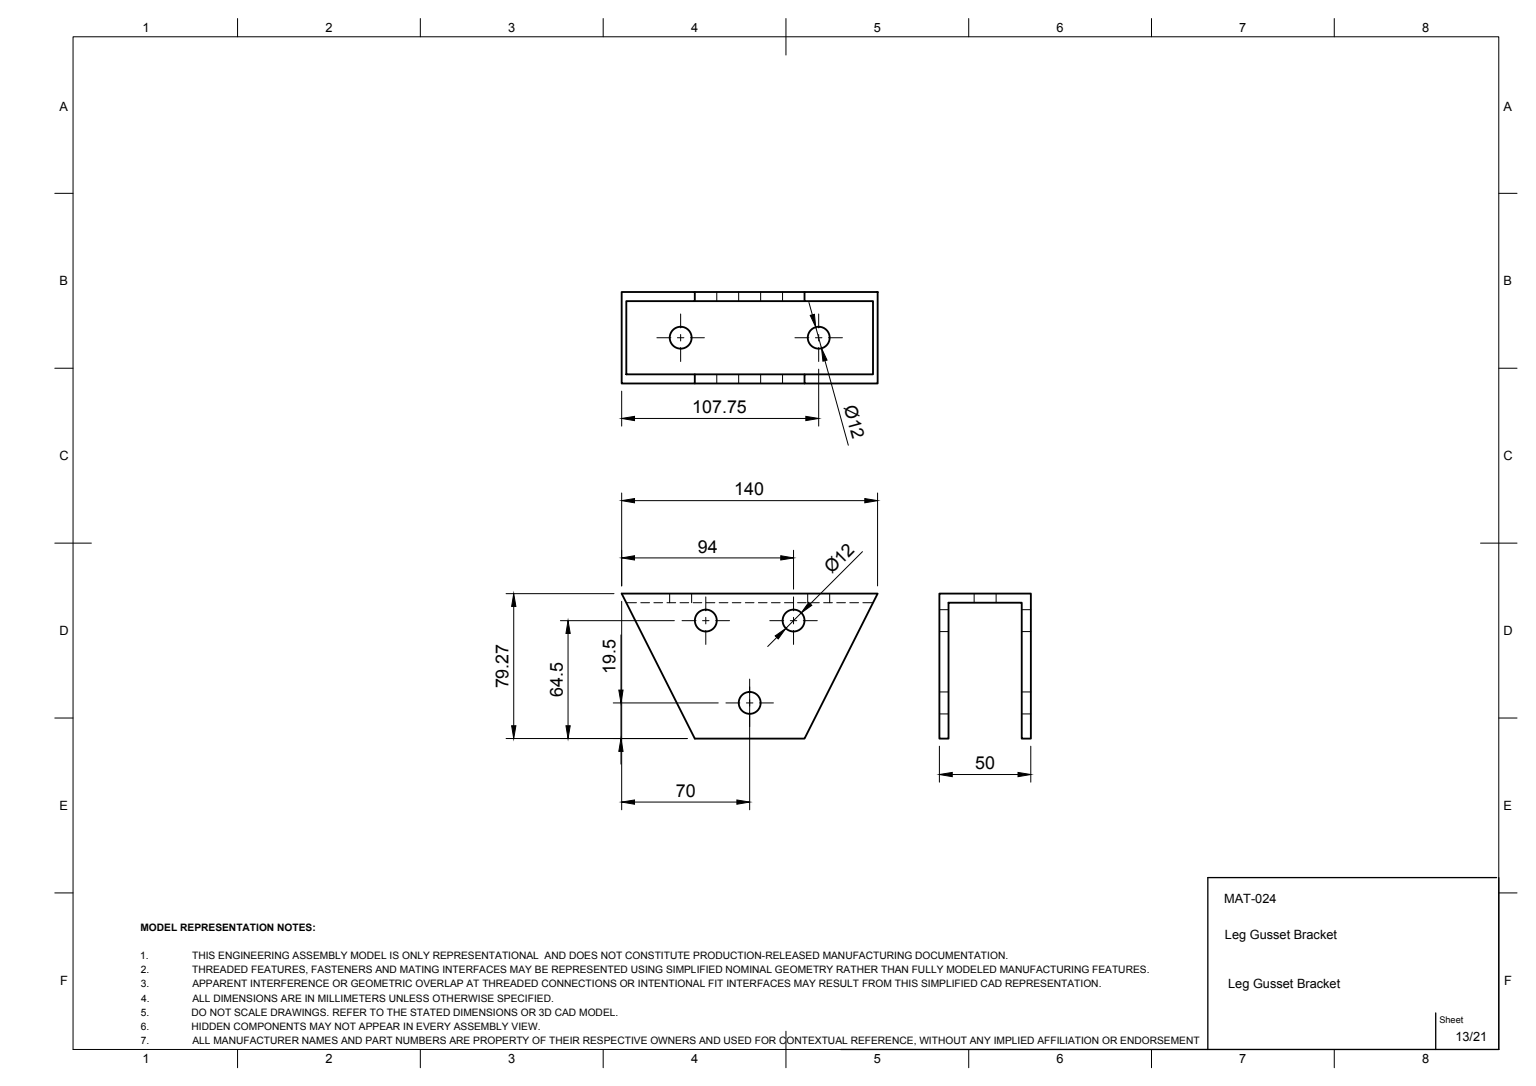
ISO-10303-21;
HEADER;
/* Generated by software containing ST-Developer
 * from STEP Tools, Inc. (www.steptools.com) 
 */

FILE_DESCRIPTION(
/* description */ ('STEP AP214'),
/* implementation_level */ '2;1');

FILE_NAME(
/* name */ 'Leg Gusset Bracket.step',
/* time_stamp */ '2026-11-14T06:34:07-08:00',
/* author */ (''),
/* organization */ (''),
/* preprocessor_version */ 'ST-DEVELOPER v20.2',
/* originating_system */ 'Autodesk Translation Framework v15.17.0.0',
/* authorisation */ '');

FILE_SCHEMA (('AUTOMOTIVE_DESIGN { 1 0 10303 214 3 1 1 }'));
ENDSEC;

DATA;
#10=MECHANICAL_DESIGN_GEOMETRIC_PRESENTATION_REPRESENTATION('',(#7320),#310623);
#7235=SHAPE_REPRESENTATION_RELATIONSHIP('SRR','None',#310909,#7252);
#7252=ADVANCED_BREP_SHAPE_REPRESENTATION('',(#7387),#310618);
#7320=STYLED_ITEM('',(#311004),#7387);
#7387=MANIFOLD_SOLID_BREP('Body1',#93771);
#7676=FACE_BOUND('',#20280,.T.);
#7677=FACE_BOUND('',#20281,.T.);
#7678=FACE_BOUND('',#20283,.T.);
#7679=FACE_BOUND('',#20284,.T.);
#7680=FACE_BOUND('',#20285,.T.);
#7681=FACE_BOUND('',#20287,.T.);
#7682=FACE_BOUND('',#20288,.T.);
#7683=FACE_BOUND('',#20289,.T.);
#7684=FACE_BOUND('',#20291,.T.);
#7685=FACE_BOUND('',#20292,.T.);
#7686=FACE_BOUND('',#20293,.T.);
#7687=FACE_BOUND('',#20295,.T.);
#7688=FACE_BOUND('',#20296,.T.);
#7689=FACE_BOUND('',#20298,.T.);
#7690=FACE_BOUND('',#20299,.T.);
#7691=FACE_BOUND('',#20300,.T.);
#8632=PLANE('',#104587);
#8633=PLANE('',#104588);
#8634=PLANE('',#104589);
#8635=PLANE('',#104590);
#8636=PLANE('',#104591);
#8637=PLANE('',#104592);
#8638=PLANE('',#104593);
#8639=PLANE('',#104594);
#8640=PLANE('',#104595);
#8641=PLANE('',#104596);
#14243=FACE_OUTER_BOUND('',#20267,.T.);
#14244=FACE_OUTER_BOUND('',#20268,.T.);
#14245=FACE_OUTER_BOUND('',#20269,.T.);
#14246=FACE_OUTER_BOUND('',#20270,.T.);
#14247=FACE_OUTER_BOUND('',#20271,.T.);
#14248=FACE_OUTER_BOUND('',#20272,.T.);
#14249=FACE_OUTER_BOUND('',#20273,.T.);
#14250=FACE_OUTER_BOUND('',#20274,.T.);
#14251=FACE_OUTER_BOUND('',#20275,.T.);
#14252=FACE_OUTER_BOUND('',#20276,.T.);
#14253=FACE_OUTER_BOUND('',#20277,.T.);
#14254=FACE_OUTER_BOUND('',#20278,.T.);
#14255=FACE_OUTER_BOUND('',#20279,.T.);
#14256=FACE_OUTER_BOUND('',#20282,.T.);
#14257=FACE_OUTER_BOUND('',#20286,.T.);
#14258=FACE_OUTER_BOUND('',#20290,.T.);
#14259=FACE_OUTER_BOUND('',#20294,.T.);
#14260=FACE_OUTER_BOUND('',#20297,.T.);
#20267=EDGE_LOOP('',(#84815,#84816,#84817,#84818));
#20268=EDGE_LOOP('',(#84819,#84820,#84821,#84822));
#20269=EDGE_LOOP('',(#84823,#84824,#84825,#84826));
#20270=EDGE_LOOP('',(#84827,#84828,#84829,#84830));
#20271=EDGE_LOOP('',(#84831,#84832,#84833,#84834));
#20272=EDGE_LOOP('',(#84835,#84836,#84837,#84838));
#20273=EDGE_LOOP('',(#84839,#84840,#84841,#84842));
#20274=EDGE_LOOP('',(#84843,#84844,#84845,#84846));
#20275=EDGE_LOOP('',(#84847,#84848,#84849,#84850,#84851,#84852,#84853,#84854));
#20276=EDGE_LOOP('',(#84855,#84856,#84857,#84858,#84859,#84860,#84861,#84862));
#20277=EDGE_LOOP('',(#84863,#84864,#84865,#84866));
#20278=EDGE_LOOP('',(#84867,#84868,#84869,#84870));
#20279=EDGE_LOOP('',(#84871,#84872,#84873,#84874));
#20280=EDGE_LOOP('',(#84875));
#20281=EDGE_LOOP('',(#84876));
#20282=EDGE_LOOP('',(#84877,#84878,#84879,#84880));
#20283=EDGE_LOOP('',(#84881));
#20284=EDGE_LOOP('',(#84882));
#20285=EDGE_LOOP('',(#84883));
#20286=EDGE_LOOP('',(#84884,#84885,#84886,#84887));
#20287=EDGE_LOOP('',(#84888));
#20288=EDGE_LOOP('',(#84889));
#20289=EDGE_LOOP('',(#84890));
#20290=EDGE_LOOP('',(#84891,#84892,#84893,#84894));
#20291=EDGE_LOOP('',(#84895));
#20292=EDGE_LOOP('',(#84896));
#20293=EDGE_LOOP('',(#84897));
#20294=EDGE_LOOP('',(#84898,#84899,#84900,#84901));
#20295=EDGE_LOOP('',(#84902));
#20296=EDGE_LOOP('',(#84903));
#20297=EDGE_LOOP('',(#84904,#84905,#84906,#84907));
#20298=EDGE_LOOP('',(#84908));
#20299=EDGE_LOOP('',(#84909));
#20300=EDGE_LOOP('',(#84910));
#24640=LINE('',#302816,#28987);
#24641=LINE('',#302822,#28988);
#24642=LINE('',#302828,#28989);
#24643=LINE('',#302834,#28990);
#24644=LINE('',#302840,#28991);
#24645=LINE('',#302846,#28992);
#24646=LINE('',#302852,#28993);
#24647=LINE('',#302858,#28994);
#24648=LINE('',#302863,#28995);
#24649=LINE('',#302865,#28996);
#24650=LINE('',#302867,#28997);
#24651=LINE('',#302869,#28998);
#24652=LINE('',#302871,#28999);
#24653=LINE('',#302873,#29000);
#24654=LINE('',#302875,#29001);
#24655=LINE('',#302876,#29002);
#24656=LINE('',#302880,#29003);
#24657=LINE('',#302882,#29004);
#24658=LINE('',#302884,#29005);
#24659=LINE('',#302886,#29006);
#24660=LINE('',#302888,#29007);
#24661=LINE('',#302890,#29008);
#24662=LINE('',#302892,#29009);
#24663=LINE('',#302893,#29010);
#24664=LINE('',#302895,#29011);
#24665=LINE('',#302896,#29012);
#24666=LINE('',#302898,#29013);
#24667=LINE('',#302899,#29014);
#24668=LINE('',#302901,#29015);
#24669=LINE('',#302902,#29016);
#24670=LINE('',#302906,#29017);
#24671=LINE('',#302908,#29018);
#28987=VECTOR('',#130227,6.00000000000001);
#28988=VECTOR('',#130234,6.00000000000001);
#28989=VECTOR('',#130241,6.00000000000001);
#28990=VECTOR('',#130248,6.00000000000001);
#28991=VECTOR('',#130255,6.00000000000001);
#28992=VECTOR('',#130262,6.00000000000001);
#28993=VECTOR('',#130269,6.00000000000001);
#28994=VECTOR('',#130276,6.00000000000001);
#28995=VECTOR('',#130281,1000.);
#28996=VECTOR('',#130282,1000.);
#28997=VECTOR('',#130283,1000.);
#28998=VECTOR('',#130284,1000.);
#28999=VECTOR('',#130285,1000.);
#29000=VECTOR('',#130286,1000.);
#29001=VECTOR('',#130287,1000.);
#29002=VECTOR('',#130288,1000.);
#29003=VECTOR('',#130291,1000.);
#29004=VECTOR('',#130292,1000.);
#29005=VECTOR('',#130293,1000.);
#29006=VECTOR('',#130294,1000.);
#29007=VECTOR('',#130295,1000.);
#29008=VECTOR('',#130296,1000.);
#29009=VECTOR('',#130297,1000.);
#29010=VECTOR('',#130298,1000.);
#29011=VECTOR('',#130301,1000.);
#29012=VECTOR('',#130302,1000.);
#29013=VECTOR('',#130305,1000.);
#29014=VECTOR('',#130306,1000.);
#29015=VECTOR('',#130309,1000.);
#29016=VECTOR('',#130310,1000.);
#29017=VECTOR('',#130317,1000.);
#29018=VECTOR('',#130320,1000.);
#35041=CIRCLE('',#104564,6.00000000000001);
#35042=CIRCLE('',#104565,6.00000000000001);
#35043=CIRCLE('',#104567,6.00000000000001);
#35044=CIRCLE('',#104568,6.00000000000001);
#35045=CIRCLE('',#104570,5.99999999999999);
#35046=CIRCLE('',#104571,6.00000000000001);
#35047=CIRCLE('',#104573,5.99999999999999);
#35048=CIRCLE('',#104574,6.00000000000001);
#35049=CIRCLE('',#104576,5.99999999999999);
#35050=CIRCLE('',#104577,6.00000000000001);
#35051=CIRCLE('',#104579,6.00000000000001);
#35052=CIRCLE('',#104580,6.00000000000001);
#35053=CIRCLE('',#104582,6.00000000000001);
#35054=CIRCLE('',#104583,6.00000000000001);
#35055=CIRCLE('',#104585,6.00000000000001);
#35056=CIRCLE('',#104586,6.00000000000001);
#43306=VERTEX_POINT('',#302813);
#43307=VERTEX_POINT('',#302815);
#43308=VERTEX_POINT('',#302819);
#43309=VERTEX_POINT('',#302821);
#43310=VERTEX_POINT('',#302825);
#43311=VERTEX_POINT('',#302827);
#43312=VERTEX_POINT('',#302831);
#43313=VERTEX_POINT('',#302833);
#43314=VERTEX_POINT('',#302837);
#43315=VERTEX_POINT('',#302839);
#43316=VERTEX_POINT('',#302843);
#43317=VERTEX_POINT('',#302845);
#43318=VERTEX_POINT('',#302849);
#43319=VERTEX_POINT('',#302851);
#43320=VERTEX_POINT('',#302855);
#43321=VERTEX_POINT('',#302857);
#43322=VERTEX_POINT('',#302861);
#43323=VERTEX_POINT('',#302862);
#43324=VERTEX_POINT('',#302864);
#43325=VERTEX_POINT('',#302866);
#43326=VERTEX_POINT('',#302868);
#43327=VERTEX_POINT('',#302870);
#43328=VERTEX_POINT('',#302872);
#43329=VERTEX_POINT('',#302874);
#43330=VERTEX_POINT('',#302878);
#43331=VERTEX_POINT('',#302879);
#43332=VERTEX_POINT('',#302881);
#43333=VERTEX_POINT('',#302883);
#43334=VERTEX_POINT('',#302885);
#43335=VERTEX_POINT('',#302887);
#43336=VERTEX_POINT('',#302889);
#43337=VERTEX_POINT('',#302891);
#57187=EDGE_CURVE('',#43306,#43306,#35041,.T.);
#57188=EDGE_CURVE('',#43306,#43307,#24640,.T.);
#57189=EDGE_CURVE('',#43307,#43307,#35042,.T.);
#57190=EDGE_CURVE('',#43308,#43308,#35043,.T.);
#57191=EDGE_CURVE('',#43308,#43309,#24641,.T.);
#57192=EDGE_CURVE('',#43309,#43309,#35044,.T.);
#57193=EDGE_CURVE('',#43310,#43310,#35045,.T.);
#57194=EDGE_CURVE('',#43310,#43311,#24642,.T.);
#57195=EDGE_CURVE('',#43311,#43311,#35046,.T.);
#57196=EDGE_CURVE('',#43312,#43312,#35047,.T.);
#57197=EDGE_CURVE('',#43312,#43313,#24643,.T.);
#57198=EDGE_CURVE('',#43313,#43313,#35048,.T.);
#57199=EDGE_CURVE('',#43314,#43314,#35049,.T.);
#57200=EDGE_CURVE('',#43314,#43315,#24644,.T.);
#57201=EDGE_CURVE('',#43315,#43315,#35050,.T.);
#57202=EDGE_CURVE('',#43316,#43316,#35051,.T.);
#57203=EDGE_CURVE('',#43316,#43317,#24645,.T.);
#57204=EDGE_CURVE('',#43317,#43317,#35052,.T.);
#57205=EDGE_CURVE('',#43318,#43318,#35053,.T.);
#57206=EDGE_CURVE('',#43318,#43319,#24646,.T.);
#57207=EDGE_CURVE('',#43319,#43319,#35054,.T.);
#57208=EDGE_CURVE('',#43320,#43320,#35055,.T.);
#57209=EDGE_CURVE('',#43320,#43321,#24647,.T.);
#57210=EDGE_CURVE('',#43321,#43321,#35056,.T.);
#57211=EDGE_CURVE('',#43322,#43323,#24648,.T.);
#57212=EDGE_CURVE('',#43323,#43324,#24649,.T.);
#57213=EDGE_CURVE('',#43324,#43325,#24650,.T.);
#57214=EDGE_CURVE('',#43326,#43325,#24651,.T.);
#57215=EDGE_CURVE('',#43327,#43326,#24652,.T.);
#57216=EDGE_CURVE('',#43327,#43328,#24653,.T.);
#57217=EDGE_CURVE('',#43328,#43329,#24654,.T.);
#57218=EDGE_CURVE('',#43329,#43322,#24655,.T.);
#57219=EDGE_CURVE('',#43330,#43331,#24656,.T.);
#57220=EDGE_CURVE('',#43330,#43332,#24657,.T.);
#57221=EDGE_CURVE('',#43332,#43333,#24658,.T.);
#57222=EDGE_CURVE('',#43333,#43334,#24659,.T.);
#57223=EDGE_CURVE('',#43335,#43334,#24660,.T.);
#57224=EDGE_CURVE('',#43335,#43336,#24661,.T.);
#57225=EDGE_CURVE('',#43336,#43337,#24662,.T.);
#57226=EDGE_CURVE('',#43331,#43337,#24663,.T.);
#57227=EDGE_CURVE('',#43324,#43330,#24664,.T.);
#57228=EDGE_CURVE('',#43325,#43331,#24665,.T.);
#57229=EDGE_CURVE('',#43334,#43329,#24666,.T.);
#57230=EDGE_CURVE('',#43328,#43335,#24667,.T.);
#57231=EDGE_CURVE('',#43337,#43326,#24668,.T.);
#57232=EDGE_CURVE('',#43336,#43327,#24669,.T.);
#57233=EDGE_CURVE('',#43323,#43332,#24670,.T.);
#57234=EDGE_CURVE('',#43322,#43333,#24671,.T.);
#84815=ORIENTED_EDGE('',*,*,#57187,.F.);
#84816=ORIENTED_EDGE('',*,*,#57188,.T.);
#84817=ORIENTED_EDGE('',*,*,#57189,.T.);
#84818=ORIENTED_EDGE('',*,*,#57188,.F.);
#84819=ORIENTED_EDGE('',*,*,#57190,.F.);
#84820=ORIENTED_EDGE('',*,*,#57191,.T.);
#84821=ORIENTED_EDGE('',*,*,#57192,.T.);
#84822=ORIENTED_EDGE('',*,*,#57191,.F.);
#84823=ORIENTED_EDGE('',*,*,#57193,.T.);
#84824=ORIENTED_EDGE('',*,*,#57194,.T.);
#84825=ORIENTED_EDGE('',*,*,#57195,.T.);
#84826=ORIENTED_EDGE('',*,*,#57194,.F.);
#84827=ORIENTED_EDGE('',*,*,#57196,.T.);
#84828=ORIENTED_EDGE('',*,*,#57197,.T.);
#84829=ORIENTED_EDGE('',*,*,#57198,.T.);
#84830=ORIENTED_EDGE('',*,*,#57197,.F.);
#84831=ORIENTED_EDGE('',*,*,#57199,.T.);
#84832=ORIENTED_EDGE('',*,*,#57200,.T.);
#84833=ORIENTED_EDGE('',*,*,#57201,.T.);
#84834=ORIENTED_EDGE('',*,*,#57200,.F.);
#84835=ORIENTED_EDGE('',*,*,#57202,.F.);
#84836=ORIENTED_EDGE('',*,*,#57203,.T.);
#84837=ORIENTED_EDGE('',*,*,#57204,.T.);
#84838=ORIENTED_EDGE('',*,*,#57203,.F.);
#84839=ORIENTED_EDGE('',*,*,#57205,.F.);
#84840=ORIENTED_EDGE('',*,*,#57206,.T.);
#84841=ORIENTED_EDGE('',*,*,#57207,.T.);
#84842=ORIENTED_EDGE('',*,*,#57206,.F.);
#84843=ORIENTED_EDGE('',*,*,#57208,.F.);
#84844=ORIENTED_EDGE('',*,*,#57209,.T.);
#84845=ORIENTED_EDGE('',*,*,#57210,.T.);
#84846=ORIENTED_EDGE('',*,*,#57209,.F.);
#84847=ORIENTED_EDGE('',*,*,#57211,.T.);
#84848=ORIENTED_EDGE('',*,*,#57212,.T.);
#84849=ORIENTED_EDGE('',*,*,#57213,.T.);
#84850=ORIENTED_EDGE('',*,*,#57214,.F.);
#84851=ORIENTED_EDGE('',*,*,#57215,.F.);
#84852=ORIENTED_EDGE('',*,*,#57216,.T.);
#84853=ORIENTED_EDGE('',*,*,#57217,.T.);
#84854=ORIENTED_EDGE('',*,*,#57218,.T.);
#84855=ORIENTED_EDGE('',*,*,#57219,.F.);
#84856=ORIENTED_EDGE('',*,*,#57220,.T.);
#84857=ORIENTED_EDGE('',*,*,#57221,.T.);
#84858=ORIENTED_EDGE('',*,*,#57222,.T.);
#84859=ORIENTED_EDGE('',*,*,#57223,.F.);
#84860=ORIENTED_EDGE('',*,*,#57224,.T.);
#84861=ORIENTED_EDGE('',*,*,#57225,.T.);
#84862=ORIENTED_EDGE('',*,*,#57226,.F.);
#84863=ORIENTED_EDGE('',*,*,#57213,.F.);
#84864=ORIENTED_EDGE('',*,*,#57227,.T.);
#84865=ORIENTED_EDGE('',*,*,#57219,.T.);
#84866=ORIENTED_EDGE('',*,*,#57228,.F.);
#84867=ORIENTED_EDGE('',*,*,#57223,.T.);
#84868=ORIENTED_EDGE('',*,*,#57229,.T.);
#84869=ORIENTED_EDGE('',*,*,#57217,.F.);
#84870=ORIENTED_EDGE('',*,*,#57230,.T.);
#84871=ORIENTED_EDGE('',*,*,#57231,.F.);
#84872=ORIENTED_EDGE('',*,*,#57225,.F.);
#84873=ORIENTED_EDGE('',*,*,#57232,.T.);
#84874=ORIENTED_EDGE('',*,*,#57215,.T.);
#84875=ORIENTED_EDGE('',*,*,#57187,.T.);
#84876=ORIENTED_EDGE('',*,*,#57190,.T.);
#84877=ORIENTED_EDGE('',*,*,#57216,.F.);
#84878=ORIENTED_EDGE('',*,*,#57232,.F.);
#84879=ORIENTED_EDGE('',*,*,#57224,.F.);
#84880=ORIENTED_EDGE('',*,*,#57230,.F.);
#84881=ORIENTED_EDGE('',*,*,#57202,.T.);
#84882=ORIENTED_EDGE('',*,*,#57205,.T.);
#84883=ORIENTED_EDGE('',*,*,#57208,.T.);
#84884=ORIENTED_EDGE('',*,*,#57214,.T.);
#84885=ORIENTED_EDGE('',*,*,#57228,.T.);
#84886=ORIENTED_EDGE('',*,*,#57226,.T.);
#84887=ORIENTED_EDGE('',*,*,#57231,.T.);
#84888=ORIENTED_EDGE('',*,*,#57195,.F.);
#84889=ORIENTED_EDGE('',*,*,#57198,.F.);
#84890=ORIENTED_EDGE('',*,*,#57201,.F.);
#84891=ORIENTED_EDGE('',*,*,#57233,.T.);
#84892=ORIENTED_EDGE('',*,*,#57220,.F.);
#84893=ORIENTED_EDGE('',*,*,#57227,.F.);
#84894=ORIENTED_EDGE('',*,*,#57212,.F.);
#84895=ORIENTED_EDGE('',*,*,#57193,.F.);
#84896=ORIENTED_EDGE('',*,*,#57196,.F.);
#84897=ORIENTED_EDGE('',*,*,#57199,.F.);
#84898=ORIENTED_EDGE('',*,*,#57234,.T.);
#84899=ORIENTED_EDGE('',*,*,#57221,.F.);
#84900=ORIENTED_EDGE('',*,*,#57233,.F.);
#84901=ORIENTED_EDGE('',*,*,#57211,.F.);
#84902=ORIENTED_EDGE('',*,*,#57189,.F.);
#84903=ORIENTED_EDGE('',*,*,#57192,.F.);
#84904=ORIENTED_EDGE('',*,*,#57229,.F.);
#84905=ORIENTED_EDGE('',*,*,#57222,.F.);
#84906=ORIENTED_EDGE('',*,*,#57234,.F.);
#84907=ORIENTED_EDGE('',*,*,#57218,.F.);
#84908=ORIENTED_EDGE('',*,*,#57204,.F.);
#84909=ORIENTED_EDGE('',*,*,#57207,.F.);
#84910=ORIENTED_EDGE('',*,*,#57210,.F.);
#87900=CYLINDRICAL_SURFACE('',#104563,6.00000000000001);
#87901=CYLINDRICAL_SURFACE('',#104566,6.00000000000001);
#87902=CYLINDRICAL_SURFACE('',#104569,6.00000000000001);
#87903=CYLINDRICAL_SURFACE('',#104572,6.00000000000001);
#87904=CYLINDRICAL_SURFACE('',#104575,6.00000000000001);
#87905=CYLINDRICAL_SURFACE('',#104578,6.00000000000001);
#87906=CYLINDRICAL_SURFACE('',#104581,6.00000000000001);
#87907=CYLINDRICAL_SURFACE('',#104584,6.00000000000001);
#93522=ADVANCED_FACE('',(#14243),#87900,.F.);
#93523=ADVANCED_FACE('',(#14244),#87901,.F.);
#93524=ADVANCED_FACE('',(#14245),#87902,.F.);
#93525=ADVANCED_FACE('',(#14246),#87903,.F.);
#93526=ADVANCED_FACE('',(#14247),#87904,.F.);
#93527=ADVANCED_FACE('',(#14248),#87905,.F.);
#93528=ADVANCED_FACE('',(#14249),#87906,.F.);
#93529=ADVANCED_FACE('',(#14250),#87907,.F.);
#93530=ADVANCED_FACE('',(#14251),#8632,.T.);
#93531=ADVANCED_FACE('',(#14252),#8633,.T.);
#93532=ADVANCED_FACE('',(#14253),#8634,.T.);
#93533=ADVANCED_FACE('',(#14254),#8635,.T.);
#93534=ADVANCED_FACE('',(#14255,#7676,#7677),#8636,.T.);
#93535=ADVANCED_FACE('',(#14256,#7678,#7679,#7680),#8637,.T.);
#93536=ADVANCED_FACE('',(#14257,#7681,#7682,#7683),#8638,.F.);
#93537=ADVANCED_FACE('',(#14258,#7684,#7685,#7686),#8639,.T.);
#93538=ADVANCED_FACE('',(#14259,#7687,#7688),#8640,.T.);
#93539=ADVANCED_FACE('',(#14260,#7689,#7690,#7691),#8641,.T.);
#93771=CLOSED_SHELL('',(#93522,#93523,#93524,#93525,#93526,#93527,#93528,
#93529,#93530,#93531,#93532,#93533,#93534,#93535,#93536,#93537,#93538,#93539));
#104562=AXIS2_PLACEMENT_3D('',#302811,#130221,#130222);
#104563=AXIS2_PLACEMENT_3D('',#302812,#130223,#130224);
#104564=AXIS2_PLACEMENT_3D('',#302814,#130225,#130226);
#104565=AXIS2_PLACEMENT_3D('',#302817,#130228,#130229);
#104566=AXIS2_PLACEMENT_3D('',#302818,#130230,#130231);
#104567=AXIS2_PLACEMENT_3D('',#302820,#130232,#130233);
#104568=AXIS2_PLACEMENT_3D('',#302823,#130235,#130236);
#104569=AXIS2_PLACEMENT_3D('',#302824,#130237,#130238);
#104570=AXIS2_PLACEMENT_3D('',#302826,#130239,#130240);
#104571=AXIS2_PLACEMENT_3D('',#302829,#130242,#130243);
#104572=AXIS2_PLACEMENT_3D('',#302830,#130244,#130245);
#104573=AXIS2_PLACEMENT_3D('',#302832,#130246,#130247);
#104574=AXIS2_PLACEMENT_3D('',#302835,#130249,#130250);
#104575=AXIS2_PLACEMENT_3D('',#302836,#130251,#130252);
#104576=AXIS2_PLACEMENT_3D('',#302838,#130253,#130254);
#104577=AXIS2_PLACEMENT_3D('',#302841,#130256,#130257);
#104578=AXIS2_PLACEMENT_3D('',#302842,#130258,#130259);
#104579=AXIS2_PLACEMENT_3D('',#302844,#130260,#130261);
#104580=AXIS2_PLACEMENT_3D('',#302847,#130263,#130264);
#104581=AXIS2_PLACEMENT_3D('',#302848,#130265,#130266);
#104582=AXIS2_PLACEMENT_3D('',#302850,#130267,#130268);
#104583=AXIS2_PLACEMENT_3D('',#302853,#130270,#130271);
#104584=AXIS2_PLACEMENT_3D('',#302854,#130272,#130273);
#104585=AXIS2_PLACEMENT_3D('',#302856,#130274,#130275);
#104586=AXIS2_PLACEMENT_3D('',#302859,#130277,#130278);
#104587=AXIS2_PLACEMENT_3D('',#302860,#130279,#130280);
#104588=AXIS2_PLACEMENT_3D('',#302877,#130289,#130290);
#104589=AXIS2_PLACEMENT_3D('',#302894,#130299,#130300);
#104590=AXIS2_PLACEMENT_3D('',#302897,#130303,#130304);
#104591=AXIS2_PLACEMENT_3D('',#302900,#130307,#130308);
#104592=AXIS2_PLACEMENT_3D('',#302903,#130311,#130312);
#104593=AXIS2_PLACEMENT_3D('',#302904,#130313,#130314);
#104594=AXIS2_PLACEMENT_3D('',#302905,#130315,#130316);
#104595=AXIS2_PLACEMENT_3D('',#302907,#130318,#130319);
#104596=AXIS2_PLACEMENT_3D('',#302909,#130321,#130322);
#130221=DIRECTION('axis',(0.,0.,1.));
#130222=DIRECTION('refdir',(1.,0.,0.));
#130223=DIRECTION('center_axis',(0.,-1.,0.));
#130224=DIRECTION('ref_axis',(0.,0.,-1.));
#130225=DIRECTION('center_axis',(0.,-1.,0.));
#130226=DIRECTION('ref_axis',(0.,0.,-1.));
#130227=DIRECTION('',(0.,-1.,0.));
#130228=DIRECTION('center_axis',(0.,-1.,0.));
#130229=DIRECTION('ref_axis',(0.,0.,-1.));
#130230=DIRECTION('center_axis',(0.,-1.,0.));
#130231=DIRECTION('ref_axis',(0.,0.,-1.));
#130232=DIRECTION('center_axis',(0.,-1.,0.));
#130233=DIRECTION('ref_axis',(0.,0.,1.));
#130234=DIRECTION('',(0.,-1.,0.));
#130235=DIRECTION('center_axis',(0.,-1.,0.));
#130236=DIRECTION('ref_axis',(0.,0.,-1.));
#130237=DIRECTION('center_axis',(1.,0.,0.));
#130238=DIRECTION('ref_axis',(0.,0.,-1.));
#130239=DIRECTION('center_axis',(-1.,-1.40133336246657E-16,0.));
#130240=DIRECTION('ref_axis',(1.40133336246657E-16,-1.,0.));
#130241=DIRECTION('',(1.,0.,0.));
#130242=DIRECTION('center_axis',(1.,0.,0.));
#130243=DIRECTION('ref_axis',(0.,0.,-1.));
#130244=DIRECTION('center_axis',(1.,0.,0.));
#130245=DIRECTION('ref_axis',(0.,0.,-1.));
#130246=DIRECTION('center_axis',(-1.,-1.40133336246657E-16,0.));
#130247=DIRECTION('ref_axis',(1.40133336246657E-16,-1.,0.));
#130248=DIRECTION('',(1.,0.,0.));
#130249=DIRECTION('center_axis',(1.,0.,0.));
#130250=DIRECTION('ref_axis',(0.,0.,-1.));
#130251=DIRECTION('center_axis',(1.,0.,0.));
#130252=DIRECTION('ref_axis',(0.,0.,-1.));
#130253=DIRECTION('center_axis',(-1.,-1.40133336246657E-16,0.));
#130254=DIRECTION('ref_axis',(1.40133336246657E-16,-1.,0.));
#130255=DIRECTION('',(1.,0.,0.));
#130256=DIRECTION('center_axis',(1.,0.,0.));
#130257=DIRECTION('ref_axis',(0.,0.,-1.));
#130258=DIRECTION('center_axis',(1.,0.,0.));
#130259=DIRECTION('ref_axis',(0.,0.,-1.));
#130260=DIRECTION('center_axis',(1.,0.,0.));
#130261=DIRECTION('ref_axis',(0.,0.,-1.));
#130262=DIRECTION('',(1.,0.,0.));
#130263=DIRECTION('center_axis',(1.,0.,0.));
#130264=DIRECTION('ref_axis',(0.,0.,-1.));
#130265=DIRECTION('center_axis',(1.,0.,0.));
#130266=DIRECTION('ref_axis',(0.,0.,-1.));
#130267=DIRECTION('center_axis',(1.,0.,0.));
#130268=DIRECTION('ref_axis',(0.,0.,-1.));
#130269=DIRECTION('',(1.,0.,0.));
#130270=DIRECTION('center_axis',(1.,0.,0.));
#130271=DIRECTION('ref_axis',(0.,0.,-1.));
#130272=DIRECTION('center_axis',(1.,0.,0.));
#130273=DIRECTION('ref_axis',(0.,0.,-1.));
#130274=DIRECTION('center_axis',(1.,0.,0.));
#130275=DIRECTION('ref_axis',(0.,0.,-1.));
#130276=DIRECTION('',(1.,0.,0.));
#130277=DIRECTION('center_axis',(1.,0.,0.));
#130278=DIRECTION('ref_axis',(0.,0.,-1.));
#130279=DIRECTION('center_axis',(0.,-0.450478595617232,0.892787228230068));
#130280=DIRECTION('ref_axis',(0.,-0.892787228230068,-0.450478595617232));
#130281=DIRECTION('',(1.,0.,0.));
#130282=DIRECTION('',(1.25109252850285E-16,-0.892787228230068,-0.450478595617232));
#130283=DIRECTION('',(1.,0.,0.));
#130284=DIRECTION('',(0.,-0.892787228230068,-0.450478595617232));
#130285=DIRECTION('',(1.,0.,0.));
#130286=DIRECTION('',(0.,-0.892787228230068,-0.450478595617232));
#130287=DIRECTION('',(1.,0.,0.));
#130288=DIRECTION('',(0.,0.892787228230068,0.450478595617232));
#130289=DIRECTION('center_axis',(0.,-0.450478595617233,-0.892787228230067));
#130290=DIRECTION('ref_axis',(0.,0.892787228230067,-0.450478595617233));
#130291=DIRECTION('',(1.,0.,0.));
#130292=DIRECTION('',(-1.25109252850285E-16,0.892787228230067,-0.450478595617233));
#130293=DIRECTION('',(-1.,0.,0.));
#130294=DIRECTION('',(0.,-0.892787228230067,0.450478595617233));
#130295=DIRECTION('',(1.,0.,0.));
#130296=DIRECTION('',(0.,0.892787228230067,-0.450478595617233));
#130297=DIRECTION('',(1.,0.,0.));
#130298=DIRECTION('',(0.,0.892787228230067,-0.450478595617233));
#130299=DIRECTION('center_axis',(0.,-1.,-2.31296463463574E-16));
#130300=DIRECTION('ref_axis',(0.,2.31296463463574E-16,-1.));
#130301=DIRECTION('',(-3.24123450872038E-32,2.31296463463574E-16,-1.));
#130302=DIRECTION('',(0.,2.31296463463574E-16,-1.));
#130303=DIRECTION('center_axis',(0.,-1.,-2.31296463463574E-16));
#130304=DIRECTION('ref_axis',(0.,2.31296463463574E-16,-1.));
#130305=DIRECTION('',(0.,-2.31296463463574E-16,1.));
#130306=DIRECTION('',(0.,2.31296463463574E-16,-1.));
#130307=DIRECTION('center_axis',(0.,1.,1.22464679914735E-16));
#130308=DIRECTION('ref_axis',(0.,-1.22464679914735E-16,1.));
#130309=DIRECTION('',(0.,-1.22464679914735E-16,1.));
#130310=DIRECTION('',(0.,-1.22464679914735E-16,1.));
#130311=DIRECTION('center_axis',(-1.,0.,0.));
#130312=DIRECTION('ref_axis',(0.,0.,1.));
#130313=DIRECTION('center_axis',(-1.,0.,0.));
#130314=DIRECTION('ref_axis',(0.,0.,1.));
#130315=DIRECTION('center_axis',(-1.,-1.40133336246657E-16,0.));
#130316=DIRECTION('ref_axis',(1.40133336246657E-16,-1.,0.));
#130317=DIRECTION('',(0.,0.,-1.));
#130318=DIRECTION('center_axis',(0.,-1.,0.));
#130319=DIRECTION('ref_axis',(0.,0.,-1.));
#130320=DIRECTION('',(0.,0.,-1.));
#130321=DIRECTION('center_axis',(1.,0.,0.));
#130322=DIRECTION('ref_axis',(0.,0.,-1.));
#302811=CARTESIAN_POINT('',(0.,0.,0.));
#302812=CARTESIAN_POINT('Origin',(-25.,1.73472347597681E-14,703.603184599603));
#302813=CARTESIAN_POINT('',(-25.,1.73472347597681E-14,709.603184599603));
#302814=CARTESIAN_POINT('Origin',(-25.,1.73472347597681E-14,703.603184599603));
#302815=CARTESIAN_POINT('',(-25.,-5.,709.603184599603));
#302816=CARTESIAN_POINT('',(-25.,1.73472347597681E-14,709.603184599603));
#302817=CARTESIAN_POINT('Origin',(-25.,-5.,703.603184599603));
#302818=CARTESIAN_POINT('Origin',(-25.,1.73472347597681E-14,779.104914303734));
#302819=CARTESIAN_POINT('',(-25.,1.73472347597681E-14,785.104914303734));
#302820=CARTESIAN_POINT('Origin',(-25.,1.73472347597681E-14,779.104914303734));
#302821=CARTESIAN_POINT('',(-25.,-5.,785.104914303734));
#302822=CARTESIAN_POINT('',(-25.,1.73472347597681E-14,785.104914303734));
#302823=CARTESIAN_POINT('Origin',(-25.,-5.,779.104914303734));
#302824=CARTESIAN_POINT('Origin',(-50.,-14.7745526128092,765.354049451668));
#302825=CARTESIAN_POINT('',(-5.00000000000001,-14.7745526128092,771.354049451668));
#302826=CARTESIAN_POINT('Origin',(-5.,-14.7745526128092,765.354049451668));
#302827=CARTESIAN_POINT('',(8.88178419700125E-15,-14.7745526128092,771.354049451668));
#302828=CARTESIAN_POINT('',(-50.,-14.7745526128092,771.354049451668));
#302829=CARTESIAN_POINT('Origin',(0.,-14.7745526128092,765.354049451668));
#302830=CARTESIAN_POINT('Origin',(-50.,-14.7745526128092,717.354049451669));
#302831=CARTESIAN_POINT('',(-5.00000000000001,-14.7745526128092,723.354049451668));
#302832=CARTESIAN_POINT('Origin',(-5.,-14.7745526128092,717.354049451669));
#302833=CARTESIAN_POINT('',(8.88178419700125E-15,-14.7745526128092,723.354049451668));
#302834=CARTESIAN_POINT('',(-50.,-14.7745526128092,723.354049451668));
#302835=CARTESIAN_POINT('Origin',(0.,-14.7745526128092,717.354049451669));
#302836=CARTESIAN_POINT('Origin',(-50.,-59.7745526128092,741.354049451668));
#302837=CARTESIAN_POINT('',(-5.,-59.7745526128092,747.354049451668));
#302838=CARTESIAN_POINT('Origin',(-5.,-59.7745526128092,741.354049451668));
#302839=CARTESIAN_POINT('',(8.88178419700125E-15,-59.7745526128092,747.354049451668));
#302840=CARTESIAN_POINT('',(-50.,-59.7745526128092,747.354049451668));
#302841=CARTESIAN_POINT('Origin',(0.,-59.7745526128092,741.354049451668));
#302842=CARTESIAN_POINT('Origin',(-50.,-14.7745526128092,765.354049451668));
#302843=CARTESIAN_POINT('',(-50.,-14.7745526128092,771.354049451668));
#302844=CARTESIAN_POINT('Origin',(-50.,-14.7745526128092,765.354049451668));
#302845=CARTESIAN_POINT('',(-45.,-14.7745526128092,771.354049451668));
#302846=CARTESIAN_POINT('',(-50.,-14.7745526128092,771.354049451668));
#302847=CARTESIAN_POINT('Origin',(-45.,-14.7745526128092,765.354049451668));
#302848=CARTESIAN_POINT('Origin',(-50.,-14.7745526128092,717.354049451669));
#302849=CARTESIAN_POINT('',(-50.,-14.7745526128092,723.354049451668));
#302850=CARTESIAN_POINT('Origin',(-50.,-14.7745526128092,717.354049451669));
#302851=CARTESIAN_POINT('',(-45.,-14.7745526128092,723.354049451668));
#302852=CARTESIAN_POINT('',(-50.,-14.7745526128092,723.354049451668));
#302853=CARTESIAN_POINT('Origin',(-45.,-14.7745526128092,717.354049451669));
#302854=CARTESIAN_POINT('Origin',(-50.,-59.7745526128092,741.354049451668));
#302855=CARTESIAN_POINT('',(-50.,-59.7745526128092,747.354049451668));
#302856=CARTESIAN_POINT('Origin',(-50.,-59.7745526128092,741.354049451668));
#302857=CARTESIAN_POINT('',(-45.,-59.7745526128092,747.354049451668));
#302858=CARTESIAN_POINT('',(-50.,-59.7745526128092,747.354049451668));
#302859=CARTESIAN_POINT('Origin',(-45.,-59.7745526128092,741.354049451668));
#302860=CARTESIAN_POINT('Origin',(-50.,-79.2745526128092,771.354049451668));
#302861=CARTESIAN_POINT('',(-45.,-5.00000000000001,808.831171763833));
#302862=CARTESIAN_POINT('',(-5.,-5.,808.831171763833));
#302863=CARTESIAN_POINT('',(-50.,-5.,808.831171763833));
#302864=CARTESIAN_POINT('',(-4.99999999999999,-79.2745526128092,771.354049451668));
#302865=CARTESIAN_POINT('',(-4.99999999999999,-79.2745526128092,771.354049451668));
#302866=CARTESIAN_POINT('',(0.,-79.2745526128092,771.354049451668));
#302867=CARTESIAN_POINT('',(-50.,-79.2745526128092,771.354049451668));
#302868=CARTESIAN_POINT('',(0.,0.,811.354049451668));
#302869=CARTESIAN_POINT('',(0.,-79.2745526128092,771.354049451668));
#302870=CARTESIAN_POINT('',(-50.,0.,811.354049451668));
#302871=CARTESIAN_POINT('',(-50.,0.,811.354049451668));
#302872=CARTESIAN_POINT('',(-50.,-79.2745526128092,771.354049451668));
#302873=CARTESIAN_POINT('',(-50.,-79.2745526128092,771.354049451668));
#302874=CARTESIAN_POINT('',(-45.,-79.2745526128092,771.354049451668));
#302875=CARTESIAN_POINT('',(-50.,-79.2745526128092,771.354049451668));
#302876=CARTESIAN_POINT('',(-45.,-79.2745526128092,771.354049451668));
#302877=CARTESIAN_POINT('Origin',(-50.,1.71450551880629E-14,671.354049451668));
#302878=CARTESIAN_POINT('',(-4.99999999999999,-79.2745526128092,711.354049451668));
#302879=CARTESIAN_POINT('',(0.,-79.2745526128092,711.354049451668));
#302880=CARTESIAN_POINT('',(-50.,-79.2745526128092,711.354049451668));
#302881=CARTESIAN_POINT('',(-5.,-5.,673.876927139504));
#302882=CARTESIAN_POINT('',(-5.,2.21713726265793E-14,671.354049451668));
#302883=CARTESIAN_POINT('',(-45.,-5.,673.876927139504));
#302884=CARTESIAN_POINT('',(-50.,-5.,673.876927139504));
#302885=CARTESIAN_POINT('',(-45.,-79.2745526128092,711.354049451668));
#302886=CARTESIAN_POINT('',(-45.,1.71450551880629E-14,671.354049451668));
#302887=CARTESIAN_POINT('',(-50.,-79.2745526128092,711.354049451668));
#302888=CARTESIAN_POINT('',(-50.,-79.2745526128092,711.354049451668));
#302889=CARTESIAN_POINT('',(-50.,1.71450551880629E-14,671.354049451668));
#302890=CARTESIAN_POINT('',(-50.,1.71450551880629E-14,671.354049451668));
#302891=CARTESIAN_POINT('',(0.,1.71450551880629E-14,671.354049451668));
#302892=CARTESIAN_POINT('',(-50.,1.71450551880629E-14,671.354049451668));
#302893=CARTESIAN_POINT('',(0.,1.71450551880629E-14,671.354049451668));
#302894=CARTESIAN_POINT('Origin',(-50.,-79.2745526128092,711.354049451668));
#302895=CARTESIAN_POINT('',(-4.99999999999999,-79.2745526128092,711.354049451668));
#302896=CARTESIAN_POINT('',(0.,-79.2745526128092,711.354049451668));
#302897=CARTESIAN_POINT('Origin',(-50.,-79.2745526128092,711.354049451668));
#302898=CARTESIAN_POINT('',(-45.,-79.2745526128092,711.354049451668));
#302899=CARTESIAN_POINT('',(-50.,-79.2745526128092,711.354049451668));
#302900=CARTESIAN_POINT('Origin',(-50.,0.,811.354049451668));
#302901=CARTESIAN_POINT('',(0.,0.,811.354049451668));
#302902=CARTESIAN_POINT('',(-50.,0.,811.354049451668));
#302903=CARTESIAN_POINT('Origin',(-50.,0.,0.));
#302904=CARTESIAN_POINT('Origin',(0.,0.,0.));
#302905=CARTESIAN_POINT('Origin',(-5.,-5.,671.354049451668));
#302906=CARTESIAN_POINT('',(-5.,-5.,671.354049451668));
#302907=CARTESIAN_POINT('Origin',(-45.,-5.,671.354049451668));
#302908=CARTESIAN_POINT('',(-45.,-5.,671.354049451668));
#302909=CARTESIAN_POINT('Origin',(-45.,-79.2745526128092,671.354049451668));
#310596=UNCERTAINTY_MEASURE_WITH_UNIT(LENGTH_MEASURE(0.01),#310624,
'DISTANCE_ACCURACY_VALUE',
'Maximum model space distance between geometric entities at asserted c
onnectivities');
#310601=UNCERTAINTY_MEASURE_WITH_UNIT(LENGTH_MEASURE(0.01),#310624,
'DISTANCE_ACCURACY_VALUE',
'Maximum model space distance between geometric entities at asserted c
onnectivities');
#310618=(
GEOMETRIC_REPRESENTATION_CONTEXT(3)
GLOBAL_UNCERTAINTY_ASSIGNED_CONTEXT((#310596))
GLOBAL_UNIT_ASSIGNED_CONTEXT((#310624,#310626,#310627))
REPRESENTATION_CONTEXT('','3D')
);
#310623=(
GEOMETRIC_REPRESENTATION_CONTEXT(3)
GLOBAL_UNCERTAINTY_ASSIGNED_CONTEXT((#310601))
GLOBAL_UNIT_ASSIGNED_CONTEXT((#310624,#310626,#310627))
REPRESENTATION_CONTEXT('','3D')
);
#310624=(
LENGTH_UNIT()
NAMED_UNIT(*)
SI_UNIT(.MILLI.,.METRE.)
);
#310626=(
NAMED_UNIT(*)
PLANE_ANGLE_UNIT()
SI_UNIT($,.RADIAN.)
);
#310627=(
NAMED_UNIT(*)
SI_UNIT($,.STERADIAN.)
SOLID_ANGLE_UNIT()
);
#310644=SHAPE_DEFINITION_REPRESENTATION(#310803,#310909);
#310803=PRODUCT_DEFINITION_SHAPE('',$,#310931);
#310909=SHAPE_REPRESENTATION('',(#104562),#310618);
#310914=PRODUCT_DEFINITION_CONTEXT('part definition',#310979,'design');
#310931=PRODUCT_DEFINITION('Leg Gusset Bracket','Leg Gusset Bracket',#310952,
#310914);
#310952=PRODUCT_DEFINITION_FORMATION('',$,#310997);
#310979=APPLICATION_CONTEXT(
'Core Data for Automotive Mechanical Design Process');
#310980=PRODUCT_CONTEXT('part definition',#310979,'mechanical');
#310997=PRODUCT('Leg Gusset Bracket','Leg Gusset Bracket',$,(#310980));
#311004=PRESENTATION_STYLE_ASSIGNMENT((#311011));
#311011=SURFACE_STYLE_USAGE(.BOTH.,#311018);
#311018=SURFACE_SIDE_STYLE('',(#311025));
#311025=SURFACE_STYLE_FILL_AREA(#311032);
#311032=FILL_AREA_STYLE('Opaque(227,224,212)',(#311039));
#311039=FILL_AREA_STYLE_COLOUR('Opaque(227,224,212)',#311046);
#311046=COLOUR_RGB('Opaque(227,224,212)',0.890196078431372,0.87843137254902,
0.831372549019608);
ENDSEC;
END-ISO-10303-21;
